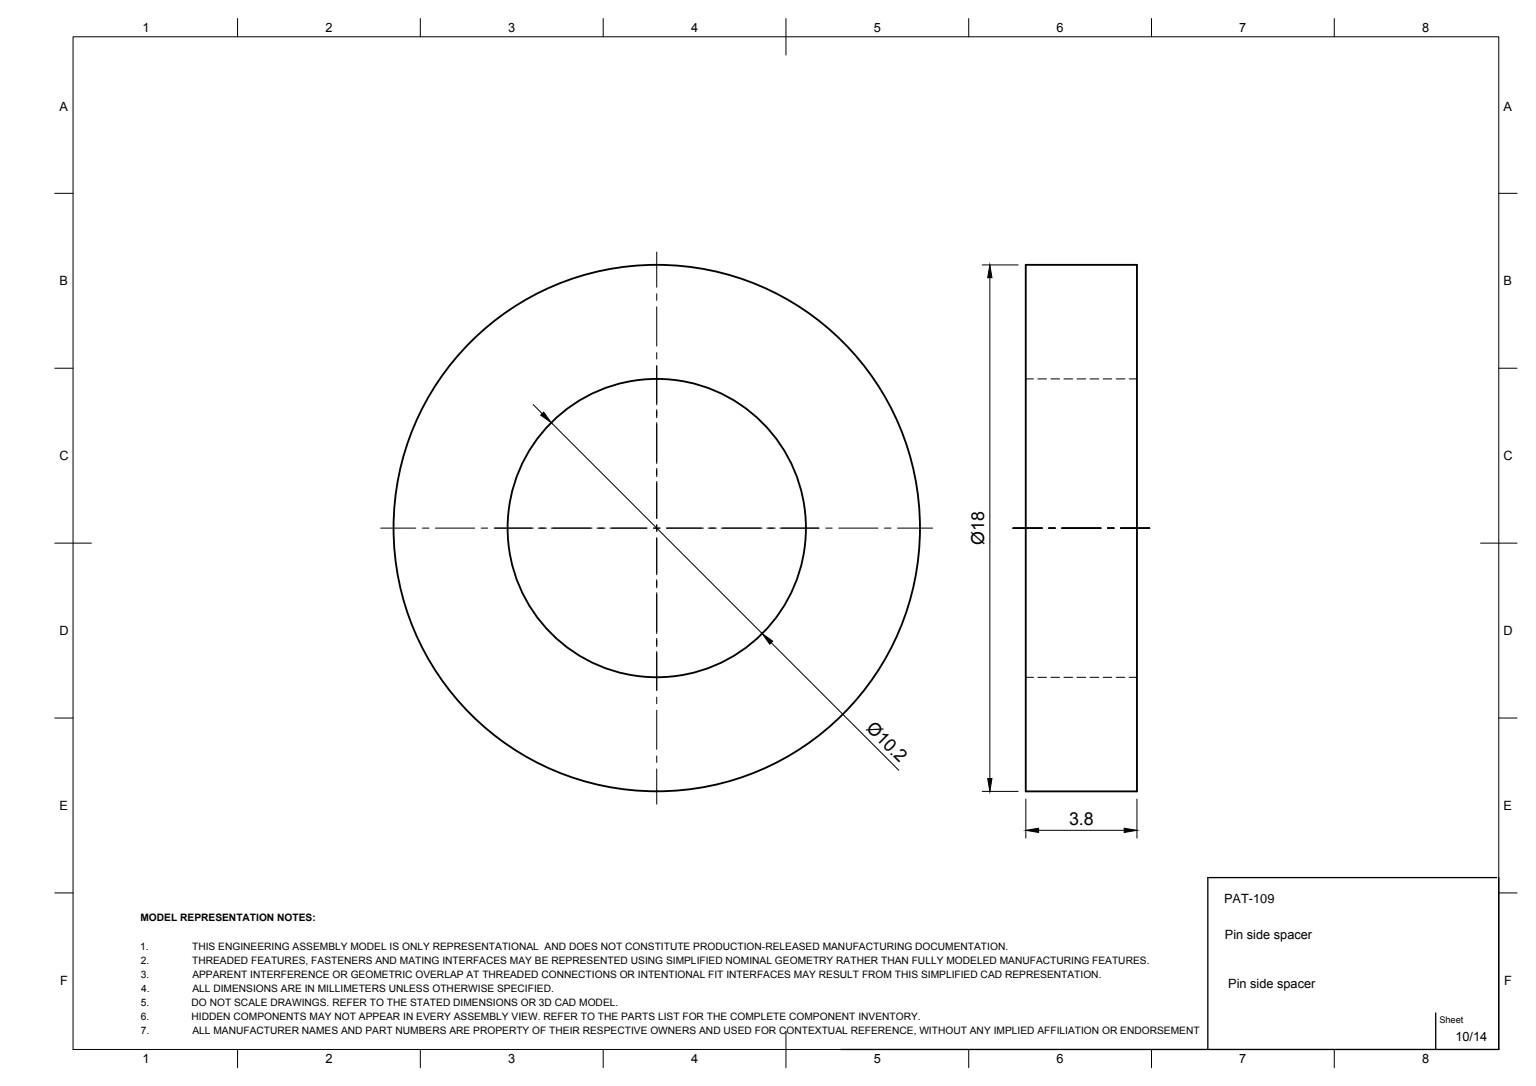
ISO-10303-21;
HEADER;
/* Generated by software containing ST-Developer
 * from STEP Tools, Inc. (www.steptools.com) 
 */

FILE_DESCRIPTION(
/* description */ ('Twin-shackle spreader bar'),
/* implementation_level */ '2;1');

FILE_NAME(
/* name */ 'Pin side spacer.step',
/* time_stamp */ '2026-10-27T20:18:10-07:00',
/* author */ (''),
/* organization */ (''),
/* preprocessor_version */ 'ST-DEVELOPER v20.2',
/* originating_system */ 'Autodesk Translation Framework v15.17.0.0',
/* authorisation */ '');

FILE_SCHEMA (('AUTOMOTIVE_DESIGN { 1 0 10303 214 3 1 1 }'));
ENDSEC;

DATA;
#10=MECHANICAL_DESIGN_GEOMETRIC_PRESENTATION_REPRESENTATION('',(#160),#1829);
#112=CIRCLE('',#1072,0.510000000000002);
#113=CIRCLE('',#1073,0.510000000000002);
#114=CIRCLE('',#1075,0.899999999999999);
#115=CIRCLE('',#1076,0.899999999999999);
#135=CYLINDRICAL_SURFACE('',#1071,0.510000000000002);
#136=CYLINDRICAL_SURFACE('',#1074,0.899999999999999);
#146=SHAPE_REPRESENTATION_RELATIONSHIP('SRR','None',#1884,#153);
#153=ADVANCED_BREP_SHAPE_REPRESENTATION('',(#167),#1825);
#160=STYLED_ITEM('',(#1984),#167);
#167=MANIFOLD_SOLID_BREP('Body1',#940);
#179=FACE_BOUND('',#276,.T.);
#180=FACE_BOUND('',#278,.T.);
#215=FACE_OUTER_BOUND('',#273,.T.);
#216=FACE_OUTER_BOUND('',#274,.T.);
#217=FACE_OUTER_BOUND('',#275,.T.);
#218=FACE_OUTER_BOUND('',#277,.T.);
#273=EDGE_LOOP('',(#772,#773,#774,#775));
#274=EDGE_LOOP('',(#776,#777,#778,#779));
#275=EDGE_LOOP('',(#780));
#276=EDGE_LOOP('',(#781));
#277=EDGE_LOOP('',(#782));
#278=EDGE_LOOP('',(#783));
#362=LINE('',#1585,#438);
#363=LINE('',#1591,#439);
#438=VECTOR('',#1294,0.510000000000002);
#439=VECTOR('',#1301,0.899999999999999);
#499=VERTEX_POINT('',#1582);
#500=VERTEX_POINT('',#1584);
#501=VERTEX_POINT('',#1588);
#502=VERTEX_POINT('',#1590);
#594=EDGE_CURVE('',#499,#499,#112,.T.);
#595=EDGE_CURVE('',#499,#500,#362,.T.);
#596=EDGE_CURVE('',#500,#500,#113,.T.);
#597=EDGE_CURVE('',#501,#501,#114,.T.);
#598=EDGE_CURVE('',#501,#502,#363,.T.);
#599=EDGE_CURVE('',#502,#502,#115,.T.);
#772=ORIENTED_EDGE('',*,*,#594,.F.);
#773=ORIENTED_EDGE('',*,*,#595,.T.);
#774=ORIENTED_EDGE('',*,*,#596,.T.);
#775=ORIENTED_EDGE('',*,*,#595,.F.);
#776=ORIENTED_EDGE('',*,*,#597,.F.);
#777=ORIENTED_EDGE('',*,*,#598,.T.);
#778=ORIENTED_EDGE('',*,*,#599,.T.);
#779=ORIENTED_EDGE('',*,*,#598,.F.);
#780=ORIENTED_EDGE('',*,*,#597,.T.);
#781=ORIENTED_EDGE('',*,*,#594,.T.);
#782=ORIENTED_EDGE('',*,*,#599,.F.);
#783=ORIENTED_EDGE('',*,*,#596,.F.);
#877=PLANE('',#1077);
#878=PLANE('',#1078);
#916=ADVANCED_FACE('',(#215),#135,.F.);
#917=ADVANCED_FACE('',(#216),#136,.T.);
#918=ADVANCED_FACE('',(#217,#179),#877,.T.);
#919=ADVANCED_FACE('',(#218,#180),#878,.F.);
#940=CLOSED_SHELL('',(#916,#917,#918,#919));
#1070=AXIS2_PLACEMENT_3D('',#1580,#1288,#1289);
#1071=AXIS2_PLACEMENT_3D('',#1581,#1290,#1291);
#1072=AXIS2_PLACEMENT_3D('',#1583,#1292,#1293);
#1073=AXIS2_PLACEMENT_3D('',#1586,#1295,#1296);
#1074=AXIS2_PLACEMENT_3D('',#1587,#1297,#1298);
#1075=AXIS2_PLACEMENT_3D('',#1589,#1299,#1300);
#1076=AXIS2_PLACEMENT_3D('',#1592,#1302,#1303);
#1077=AXIS2_PLACEMENT_3D('',#1593,#1304,#1305);
#1078=AXIS2_PLACEMENT_3D('',#1594,#1306,#1307);
#1288=DIRECTION('axis',(0.,0.,1.));
#1289=DIRECTION('refdir',(1.,0.,0.));
#1290=DIRECTION('center_axis',(0.,1.,0.));
#1291=DIRECTION('ref_axis',(1.,0.,0.));
#1292=DIRECTION('center_axis',(0.,-1.,0.));
#1293=DIRECTION('ref_axis',(1.,0.,0.));
#1294=DIRECTION('',(0.,-1.,0.));
#1295=DIRECTION('center_axis',(0.,-1.,0.));
#1296=DIRECTION('ref_axis',(1.,0.,0.));
#1297=DIRECTION('center_axis',(0.,1.,0.));
#1298=DIRECTION('ref_axis',(1.,0.,0.));
#1299=DIRECTION('center_axis',(0.,1.,0.));
#1300=DIRECTION('ref_axis',(1.,0.,0.));
#1301=DIRECTION('',(0.,-1.,0.));
#1302=DIRECTION('center_axis',(0.,1.,0.));
#1303=DIRECTION('ref_axis',(1.,0.,0.));
#1304=DIRECTION('center_axis',(0.,1.,0.));
#1305=DIRECTION('ref_axis',(1.,0.,0.));
#1306=DIRECTION('center_axis',(0.,1.,0.));
#1307=DIRECTION('ref_axis',(1.,0.,0.));
#1580=CARTESIAN_POINT('',(0.,0.,0.));
#1581=CARTESIAN_POINT('Origin',(-21.,0.61,-2.));
#1582=CARTESIAN_POINT('',(-21.51,0.99,-2.));
#1583=CARTESIAN_POINT('Origin',(-21.,0.99,-2.));
#1584=CARTESIAN_POINT('',(-21.51,0.61,-2.));
#1585=CARTESIAN_POINT('',(-21.51,0.61,-2.));
#1586=CARTESIAN_POINT('Origin',(-21.,0.61,-2.));
#1587=CARTESIAN_POINT('Origin',(-21.,0.61,-2.));
#1588=CARTESIAN_POINT('',(-21.9,0.99,-2.));
#1589=CARTESIAN_POINT('Origin',(-21.,0.99,-2.));
#1590=CARTESIAN_POINT('',(-21.9,0.61,-2.));
#1591=CARTESIAN_POINT('',(-21.9,0.61,-2.));
#1592=CARTESIAN_POINT('Origin',(-21.,0.61,-2.));
#1593=CARTESIAN_POINT('Origin',(-21.,0.99,-2.));
#1594=CARTESIAN_POINT('Origin',(-21.,0.61,-2.));
#1813=UNCERTAINTY_MEASURE_WITH_UNIT(LENGTH_MEASURE(0.001),#1830,
'DISTANCE_ACCURACY_VALUE',
'Maximum model space distance between geometric entities at asserted c
onnectivities');
#1817=UNCERTAINTY_MEASURE_WITH_UNIT(LENGTH_MEASURE(0.001),#1830,
'DISTANCE_ACCURACY_VALUE',
'Maximum model space distance between geometric entities at asserted c
onnectivities');
#1825=(
GEOMETRIC_REPRESENTATION_CONTEXT(3)
GLOBAL_UNCERTAINTY_ASSIGNED_CONTEXT((#1813))
GLOBAL_UNIT_ASSIGNED_CONTEXT((#1830,#1832,#1833))
REPRESENTATION_CONTEXT('','3D')
);
#1829=(
GEOMETRIC_REPRESENTATION_CONTEXT(3)
GLOBAL_UNCERTAINTY_ASSIGNED_CONTEXT((#1817))
GLOBAL_UNIT_ASSIGNED_CONTEXT((#1830,#1832,#1833))
REPRESENTATION_CONTEXT('','3D')
);
#1830=(
LENGTH_UNIT()
NAMED_UNIT(*)
SI_UNIT(.CENTI.,.METRE.)
);
#1832=(
NAMED_UNIT(*)
PLANE_ANGLE_UNIT()
SI_UNIT($,.RADIAN.)
);
#1833=(
NAMED_UNIT(*)
SI_UNIT($,.STERADIAN.)
SOLID_ANGLE_UNIT()
);
#1841=SHAPE_DEFINITION_REPRESENTATION(#1856,#1884);
#1856=PRODUCT_DEFINITION_SHAPE('',$,#1896);
#1884=SHAPE_REPRESENTATION('',(#1070),#1825);
#1888=PRODUCT_DEFINITION_CONTEXT('part definition',#1923,'design');
#1896=PRODUCT_DEFINITION('Pin side spacer','Pin side spacer',#1907,#1888);
#1907=PRODUCT_DEFINITION_FORMATION('',$,#1932);
#1923=APPLICATION_CONTEXT(
'Core Data for Automotive Mechanical Design Process');
#1924=PRODUCT_CONTEXT('part definition',#1923,'mechanical');
#1932=PRODUCT('Pin side spacer','Pin side spacer','Pin side spacer',(#1924));
#1978=COLOUR_RGB('Grey',0.48,0.52,0.57);
#1979=FILL_AREA_STYLE_COLOUR('',#1978);
#1980=FILL_AREA_STYLE('',(#1979));
#1981=SURFACE_STYLE_FILL_AREA(#1980);
#1982=SURFACE_SIDE_STYLE('',(#1981));
#1983=SURFACE_STYLE_USAGE(.BOTH.,#1982);
#1984=PRESENTATION_STYLE_ASSIGNMENT((#1983));
ENDSEC;
END-ISO-10303-21;
